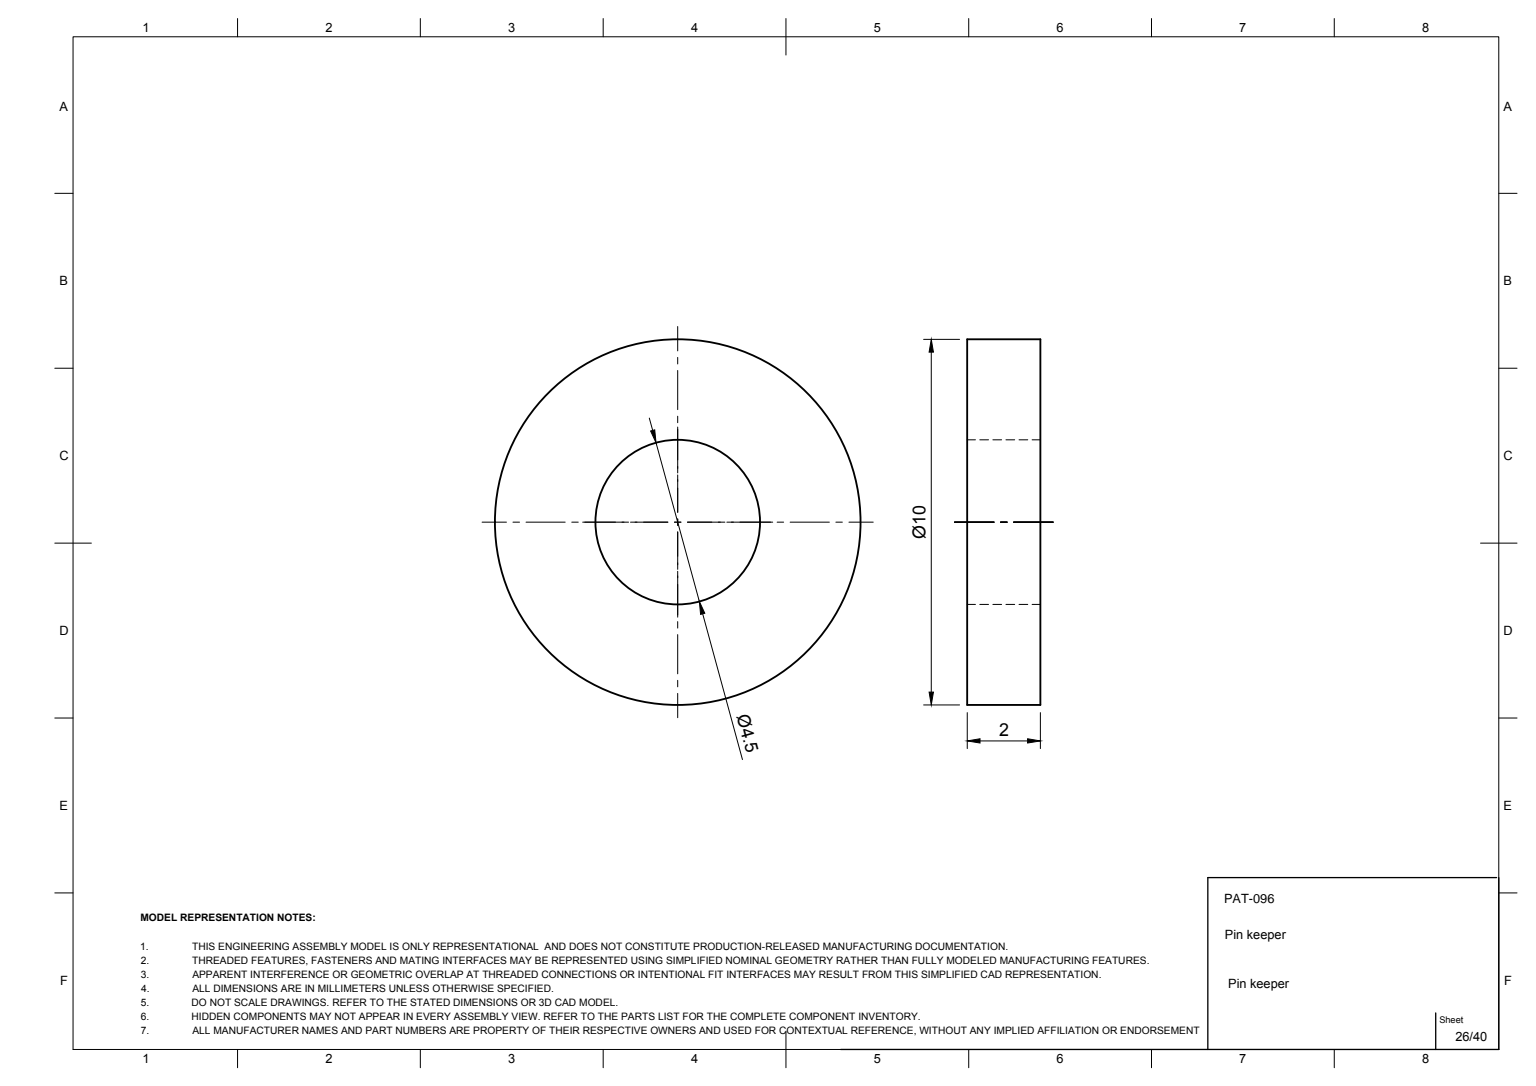
ISO-10303-21;
HEADER;
/* Generated by software containing ST-Developer
 * from STEP Tools, Inc. (www.steptools.com) 
 */

FILE_DESCRIPTION(
/* description */ ('PAT-096'),
/* implementation_level */ '2;1');

FILE_NAME(
/* name */ 'Pin keeper.step',
/* time_stamp */ '2026-10-29T17:03:14-07:00',
/* author */ (''),
/* organization */ (''),
/* preprocessor_version */ 'ST-DEVELOPER v20.2',
/* originating_system */ 'Autodesk Translation Framework v15.17.0.0',
/* authorisation */ '');

FILE_SCHEMA (('AUTOMOTIVE_DESIGN { 1 0 10303 214 3 1 1 }'));
ENDSEC;

DATA;
#10=MECHANICAL_DESIGN_GEOMETRIC_PRESENTATION_REPRESENTATION('',(#435),#10650);
#365=SHAPE_REPRESENTATION_RELATIONSHIP('SRR','None',#10830,#396);
#396=ADVANCED_BREP_SHAPE_REPRESENTATION('',(#472),#10648);
#435=STYLED_ITEM('',(#11064),#472);
#472=MANIFOLD_SOLID_BREP('Body1',#5570);
#609=FACE_BOUND('',#1581,.T.);
#610=FACE_BOUND('',#1583,.T.);
#777=PLANE('',#6592);
#778=PLANE('',#6593);
#1106=FACE_OUTER_BOUND('',#1578,.T.);
#1107=FACE_OUTER_BOUND('',#1579,.T.);
#1108=FACE_OUTER_BOUND('',#1580,.T.);
#1109=FACE_OUTER_BOUND('',#1582,.T.);
#1578=EDGE_LOOP('',(#5001,#5002,#5003,#5004));
#1579=EDGE_LOOP('',(#5005,#5006,#5007,#5008));
#1580=EDGE_LOOP('',(#5009));
#1581=EDGE_LOOP('',(#5010));
#1582=EDGE_LOOP('',(#5011));
#1583=EDGE_LOOP('',(#5012));
#1905=LINE('',#10444,#2234);
#1906=LINE('',#10450,#2235);
#2234=VECTOR('',#8321,0.225);
#2235=VECTOR('',#8328,0.5);
#2567=CIRCLE('',#6587,0.225);
#2568=CIRCLE('',#6588,0.225);
#2569=CIRCLE('',#6590,0.5);
#2570=CIRCLE('',#6591,0.5);
#3013=VERTEX_POINT('',#10441);
#3014=VERTEX_POINT('',#10443);
#3015=VERTEX_POINT('',#10447);
#3016=VERTEX_POINT('',#10449);
#3679=EDGE_CURVE('',#3013,#3013,#2567,.T.);
#3680=EDGE_CURVE('',#3013,#3014,#1905,.T.);
#3681=EDGE_CURVE('',#3014,#3014,#2568,.T.);
#3682=EDGE_CURVE('',#3015,#3015,#2569,.T.);
#3683=EDGE_CURVE('',#3015,#3016,#1906,.T.);
#3684=EDGE_CURVE('',#3016,#3016,#2570,.T.);
#5001=ORIENTED_EDGE('',*,*,#3679,.F.);
#5002=ORIENTED_EDGE('',*,*,#3680,.T.);
#5003=ORIENTED_EDGE('',*,*,#3681,.T.);
#5004=ORIENTED_EDGE('',*,*,#3680,.F.);
#5005=ORIENTED_EDGE('',*,*,#3682,.F.);
#5006=ORIENTED_EDGE('',*,*,#3683,.T.);
#5007=ORIENTED_EDGE('',*,*,#3684,.T.);
#5008=ORIENTED_EDGE('',*,*,#3683,.F.);
#5009=ORIENTED_EDGE('',*,*,#3682,.T.);
#5010=ORIENTED_EDGE('',*,*,#3679,.T.);
#5011=ORIENTED_EDGE('',*,*,#3684,.F.);
#5012=ORIENTED_EDGE('',*,*,#3681,.F.);
#5191=CYLINDRICAL_SURFACE('',#6586,0.225);
#5192=CYLINDRICAL_SURFACE('',#6589,0.5);
#5511=ADVANCED_FACE('',(#1106),#5191,.F.);
#5512=ADVANCED_FACE('',(#1107),#5192,.T.);
#5513=ADVANCED_FACE('',(#1108,#609),#777,.T.);
#5514=ADVANCED_FACE('',(#1109,#610),#778,.F.);
#5570=CLOSED_SHELL('',(#5511,#5512,#5513,#5514));
#6585=AXIS2_PLACEMENT_3D('',#10439,#8315,#8316);
#6586=AXIS2_PLACEMENT_3D('',#10440,#8317,#8318);
#6587=AXIS2_PLACEMENT_3D('',#10442,#8319,#8320);
#6588=AXIS2_PLACEMENT_3D('',#10445,#8322,#8323);
#6589=AXIS2_PLACEMENT_3D('',#10446,#8324,#8325);
#6590=AXIS2_PLACEMENT_3D('',#10448,#8326,#8327);
#6591=AXIS2_PLACEMENT_3D('',#10451,#8329,#8330);
#6592=AXIS2_PLACEMENT_3D('',#10452,#8331,#8332);
#6593=AXIS2_PLACEMENT_3D('',#10453,#8333,#8334);
#8315=DIRECTION('axis',(0.,0.,1.));
#8316=DIRECTION('refdir',(1.,0.,0.));
#8317=DIRECTION('center_axis',(0.,0.,1.));
#8318=DIRECTION('ref_axis',(1.,0.,0.));
#8319=DIRECTION('center_axis',(0.,0.,-1.));
#8320=DIRECTION('ref_axis',(1.,0.,0.));
#8321=DIRECTION('',(0.,0.,-1.));
#8322=DIRECTION('center_axis',(0.,0.,-1.));
#8323=DIRECTION('ref_axis',(1.,0.,0.));
#8324=DIRECTION('center_axis',(0.,0.,1.));
#8325=DIRECTION('ref_axis',(1.,0.,0.));
#8326=DIRECTION('center_axis',(0.,0.,1.));
#8327=DIRECTION('ref_axis',(1.,0.,0.));
#8328=DIRECTION('',(0.,0.,-1.));
#8329=DIRECTION('center_axis',(0.,0.,1.));
#8330=DIRECTION('ref_axis',(1.,0.,0.));
#8331=DIRECTION('center_axis',(0.,0.,1.));
#8332=DIRECTION('ref_axis',(1.,0.,0.));
#8333=DIRECTION('center_axis',(0.,0.,1.));
#8334=DIRECTION('ref_axis',(1.,0.,0.));
#10439=CARTESIAN_POINT('',(0.,0.,0.));
#10440=CARTESIAN_POINT('Origin',(0.,2.,10.1));
#10441=CARTESIAN_POINT('',(-0.225,2.,10.3));
#10442=CARTESIAN_POINT('Origin',(0.,2.,10.3));
#10443=CARTESIAN_POINT('',(-0.225,2.,10.1));
#10444=CARTESIAN_POINT('',(-0.225,2.,10.1));
#10445=CARTESIAN_POINT('Origin',(0.,2.,10.1));
#10446=CARTESIAN_POINT('Origin',(0.,2.,10.1));
#10447=CARTESIAN_POINT('',(-0.5,2.,10.3));
#10448=CARTESIAN_POINT('Origin',(0.,2.,10.3));
#10449=CARTESIAN_POINT('',(-0.5,2.,10.1));
#10450=CARTESIAN_POINT('',(-0.5,2.,10.1));
#10451=CARTESIAN_POINT('Origin',(0.,2.,10.1));
#10452=CARTESIAN_POINT('Origin',(0.,2.,10.3));
#10453=CARTESIAN_POINT('Origin',(0.,2.,10.1));
#10609=UNCERTAINTY_MEASURE_WITH_UNIT(LENGTH_MEASURE(0.001),#10651,
'DISTANCE_ACCURACY_VALUE',
'Maximum model space distance between geometric entities at asserted c
onnectivities');
#10611=UNCERTAINTY_MEASURE_WITH_UNIT(LENGTH_MEASURE(0.001),#10651,
'DISTANCE_ACCURACY_VALUE',
'Maximum model space distance between geometric entities at asserted c
onnectivities');
#10648=(
GEOMETRIC_REPRESENTATION_CONTEXT(3)
GLOBAL_UNCERTAINTY_ASSIGNED_CONTEXT((#10609))
GLOBAL_UNIT_ASSIGNED_CONTEXT((#10651,#10653,#10654))
REPRESENTATION_CONTEXT('','3D')
);
#10650=(
GEOMETRIC_REPRESENTATION_CONTEXT(3)
GLOBAL_UNCERTAINTY_ASSIGNED_CONTEXT((#10611))
GLOBAL_UNIT_ASSIGNED_CONTEXT((#10651,#10653,#10654))
REPRESENTATION_CONTEXT('','3D')
);
#10651=(
LENGTH_UNIT()
NAMED_UNIT(*)
SI_UNIT(.CENTI.,.METRE.)
);
#10653=(
NAMED_UNIT(*)
PLANE_ANGLE_UNIT()
SI_UNIT($,.RADIAN.)
);
#10654=(
NAMED_UNIT(*)
SI_UNIT($,.STERADIAN.)
SOLID_ANGLE_UNIT()
);
#10691=SHAPE_DEFINITION_REPRESENTATION(#10739,#10830);
#10739=PRODUCT_DEFINITION_SHAPE('',$,#10869);
#10830=SHAPE_REPRESENTATION('',(#6585),#10648);
#10832=PRODUCT_DEFINITION_CONTEXT('part definition',#10948,'design');
#10869=PRODUCT_DEFINITION('Pin keeper','Pin keeper',#10907,#10832);
#10907=PRODUCT_DEFINITION_FORMATION('',$,#10986);
#10948=APPLICATION_CONTEXT(
'Core Data for Automotive Mechanical Design Process');
#10949=PRODUCT_CONTEXT('part definition',#10948,'mechanical');
#10986=PRODUCT('Pin keeper','Pin keeper','Pin keeper',(#10949));
#11058=COLOUR_RGB('Grey',0.48,0.52,0.57);
#11059=FILL_AREA_STYLE_COLOUR('',#11058);
#11060=FILL_AREA_STYLE('',(#11059));
#11061=SURFACE_STYLE_FILL_AREA(#11060);
#11062=SURFACE_SIDE_STYLE('',(#11061));
#11063=SURFACE_STYLE_USAGE(.BOTH.,#11062);
#11064=PRESENTATION_STYLE_ASSIGNMENT((#11063));
ENDSEC;
END-ISO-10303-21;
